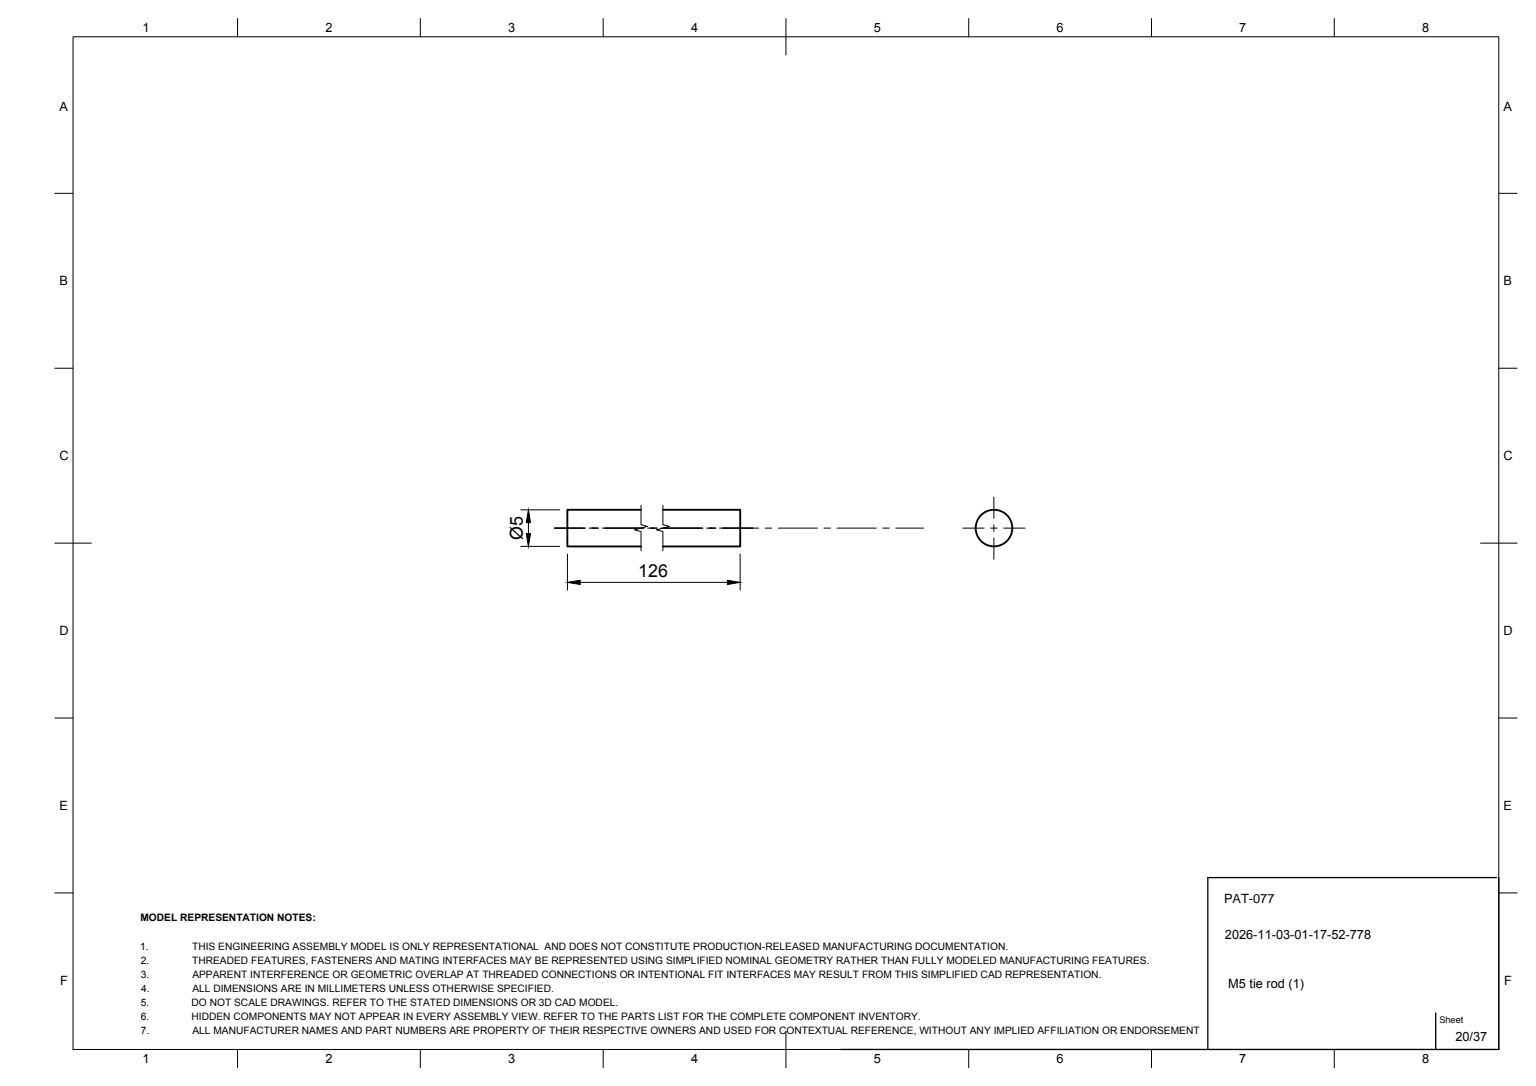
ISO-10303-21;
HEADER;
/* Generated by software containing ST-Developer
 * from STEP Tools, Inc. (www.steptools.com) 
 */

FILE_DESCRIPTION(
/* description */ ('Pallet stop with pneumatic fitting'),
/* implementation_level */ '2;1');

FILE_NAME(
/* name */ 'M5 tie rod (1).step',
/* time_stamp */ '2026-10-27T10:51:41-07:00',
/* author */ (''),
/* organization */ (''),
/* preprocessor_version */ 'ST-DEVELOPER v20.2',
/* originating_system */ 'Autodesk Translation Framework v15.17.0.0',
/* authorisation */ '');

FILE_SCHEMA (('AUTOMOTIVE_DESIGN { 1 0 10303 214 3 1 1 }'));
ENDSEC;

DATA;
#10=MECHANICAL_DESIGN_GEOMETRIC_PRESENTATION_REPRESENTATION('',(#372),#10265);
#308=SHAPE_REPRESENTATION_RELATIONSHIP('SRR','None',#10421,#340);
#340=ADVANCED_BREP_SHAPE_REPRESENTATION('',(#404),#10245);
#372=STYLED_ITEM('',(#10655),#404);
#404=MANIFOLD_SOLID_BREP('Body1',#5060);
#626=PLANE('',#5737);
#627=PLANE('',#5738);
#885=FACE_OUTER_BOUND('',#1284,.T.);
#886=FACE_OUTER_BOUND('',#1285,.T.);
#887=FACE_OUTER_BOUND('',#1286,.T.);
#1284=EDGE_LOOP('',(#3982,#3983,#3984,#3985));
#1285=EDGE_LOOP('',(#3986));
#1286=EDGE_LOOP('',(#3987));
#1633=LINE('',#9337,#1968);
#1968=VECTOR('',#6840,0.25);
#2296=CIRCLE('',#5735,0.25);
#2297=CIRCLE('',#5736,0.25);
#2596=VERTEX_POINT('',#9334);
#2597=VERTEX_POINT('',#9336);
#3090=EDGE_CURVE('',#2596,#2596,#2296,.T.);
#3091=EDGE_CURVE('',#2596,#2597,#1633,.T.);
#3092=EDGE_CURVE('',#2597,#2597,#2297,.T.);
#3982=ORIENTED_EDGE('',*,*,#3090,.F.);
#3983=ORIENTED_EDGE('',*,*,#3091,.T.);
#3984=ORIENTED_EDGE('',*,*,#3092,.T.);
#3985=ORIENTED_EDGE('',*,*,#3091,.F.);
#3986=ORIENTED_EDGE('',*,*,#3090,.T.);
#3987=ORIENTED_EDGE('',*,*,#3092,.F.);
#4689=CYLINDRICAL_SURFACE('',#5734,0.25);
#4880=ADVANCED_FACE('',(#885),#4689,.T.);
#4881=ADVANCED_FACE('',(#886),#626,.T.);
#4882=ADVANCED_FACE('',(#887),#627,.F.);
#5060=CLOSED_SHELL('',(#4880,#4881,#4882));
#5733=AXIS2_PLACEMENT_3D('',#9332,#6834,#6835);
#5734=AXIS2_PLACEMENT_3D('',#9333,#6836,#6837);
#5735=AXIS2_PLACEMENT_3D('',#9335,#6838,#6839);
#5736=AXIS2_PLACEMENT_3D('',#9338,#6841,#6842);
#5737=AXIS2_PLACEMENT_3D('',#9339,#6843,#6844);
#5738=AXIS2_PLACEMENT_3D('',#9340,#6845,#6846);
#6834=DIRECTION('axis',(0.,0.,1.));
#6835=DIRECTION('refdir',(1.,0.,0.));
#6836=DIRECTION('center_axis',(0.,0.,1.));
#6837=DIRECTION('ref_axis',(1.,0.,0.));
#6838=DIRECTION('center_axis',(0.,0.,1.));
#6839=DIRECTION('ref_axis',(1.,0.,0.));
#6840=DIRECTION('',(0.,0.,-1.));
#6841=DIRECTION('center_axis',(0.,0.,1.));
#6842=DIRECTION('ref_axis',(1.,0.,0.));
#6843=DIRECTION('center_axis',(0.,0.,1.));
#6844=DIRECTION('ref_axis',(1.,0.,0.));
#6845=DIRECTION('center_axis',(0.,0.,1.));
#6846=DIRECTION('ref_axis',(1.,0.,0.));
#9332=CARTESIAN_POINT('',(0.,0.,0.));
#9333=CARTESIAN_POINT('Origin',(2.72720779386421,5.27279220613579,-1.8));
#9334=CARTESIAN_POINT('',(2.47720779386421,5.27279220613579,10.8));
#9335=CARTESIAN_POINT('Origin',(2.72720779386421,5.27279220613579,10.8));
#9336=CARTESIAN_POINT('',(2.47720779386421,5.27279220613579,-1.8));
#9337=CARTESIAN_POINT('',(2.47720779386421,5.27279220613579,-1.8));
#9338=CARTESIAN_POINT('Origin',(2.72720779386421,5.27279220613579,-1.8));
#9339=CARTESIAN_POINT('Origin',(2.72720779386421,5.27279220613579,10.8));
#9340=CARTESIAN_POINT('Origin',(2.72720779386421,5.27279220613579,-1.8));
#10207=UNCERTAINTY_MEASURE_WITH_UNIT(LENGTH_MEASURE(0.001),#10266,
'DISTANCE_ACCURACY_VALUE',
'Maximum model space distance between geometric entities at asserted c
onnectivities');
#10227=UNCERTAINTY_MEASURE_WITH_UNIT(LENGTH_MEASURE(0.001),#10266,
'DISTANCE_ACCURACY_VALUE',
'Maximum model space distance between geometric entities at asserted c
onnectivities');
#10245=(
GEOMETRIC_REPRESENTATION_CONTEXT(3)
GLOBAL_UNCERTAINTY_ASSIGNED_CONTEXT((#10207))
GLOBAL_UNIT_ASSIGNED_CONTEXT((#10266,#10268,#10269))
REPRESENTATION_CONTEXT('','3D')
);
#10265=(
GEOMETRIC_REPRESENTATION_CONTEXT(3)
GLOBAL_UNCERTAINTY_ASSIGNED_CONTEXT((#10227))
GLOBAL_UNIT_ASSIGNED_CONTEXT((#10266,#10268,#10269))
REPRESENTATION_CONTEXT('','3D')
);
#10266=(
LENGTH_UNIT()
NAMED_UNIT(*)
SI_UNIT(.CENTI.,.METRE.)
);
#10268=(
NAMED_UNIT(*)
PLANE_ANGLE_UNIT()
SI_UNIT($,.RADIAN.)
);
#10269=(
NAMED_UNIT(*)
SI_UNIT($,.STERADIAN.)
SOLID_ANGLE_UNIT()
);
#10287=SHAPE_DEFINITION_REPRESENTATION(#10324,#10421);
#10324=PRODUCT_DEFINITION_SHAPE('',$,#10459);
#10421=SHAPE_REPRESENTATION('',(#5733),#10245);
#10441=PRODUCT_DEFINITION_CONTEXT('part definition',#10554,'design');
#10459=PRODUCT_DEFINITION('M5 tie rod (1)','M5 tie rod (1)',#10496,#10441);
#10496=PRODUCT_DEFINITION_FORMATION('',$,#10573);
#10554=APPLICATION_CONTEXT(
'Core Data for Automotive Mechanical Design Process');
#10555=PRODUCT_CONTEXT('part definition',#10554,'mechanical');
#10573=PRODUCT('M5 tie rod (1)','M5 tie rod (1)','M5 tie rod (1)',(#10555));
#10649=COLOUR_RGB('Grey',0.48,0.52,0.57);
#10650=FILL_AREA_STYLE_COLOUR('',#10649);
#10651=FILL_AREA_STYLE('',(#10650));
#10652=SURFACE_STYLE_FILL_AREA(#10651);
#10653=SURFACE_SIDE_STYLE('',(#10652));
#10654=SURFACE_STYLE_USAGE(.BOTH.,#10653);
#10655=PRESENTATION_STYLE_ASSIGNMENT((#10654));
ENDSEC;
END-ISO-10303-21;
